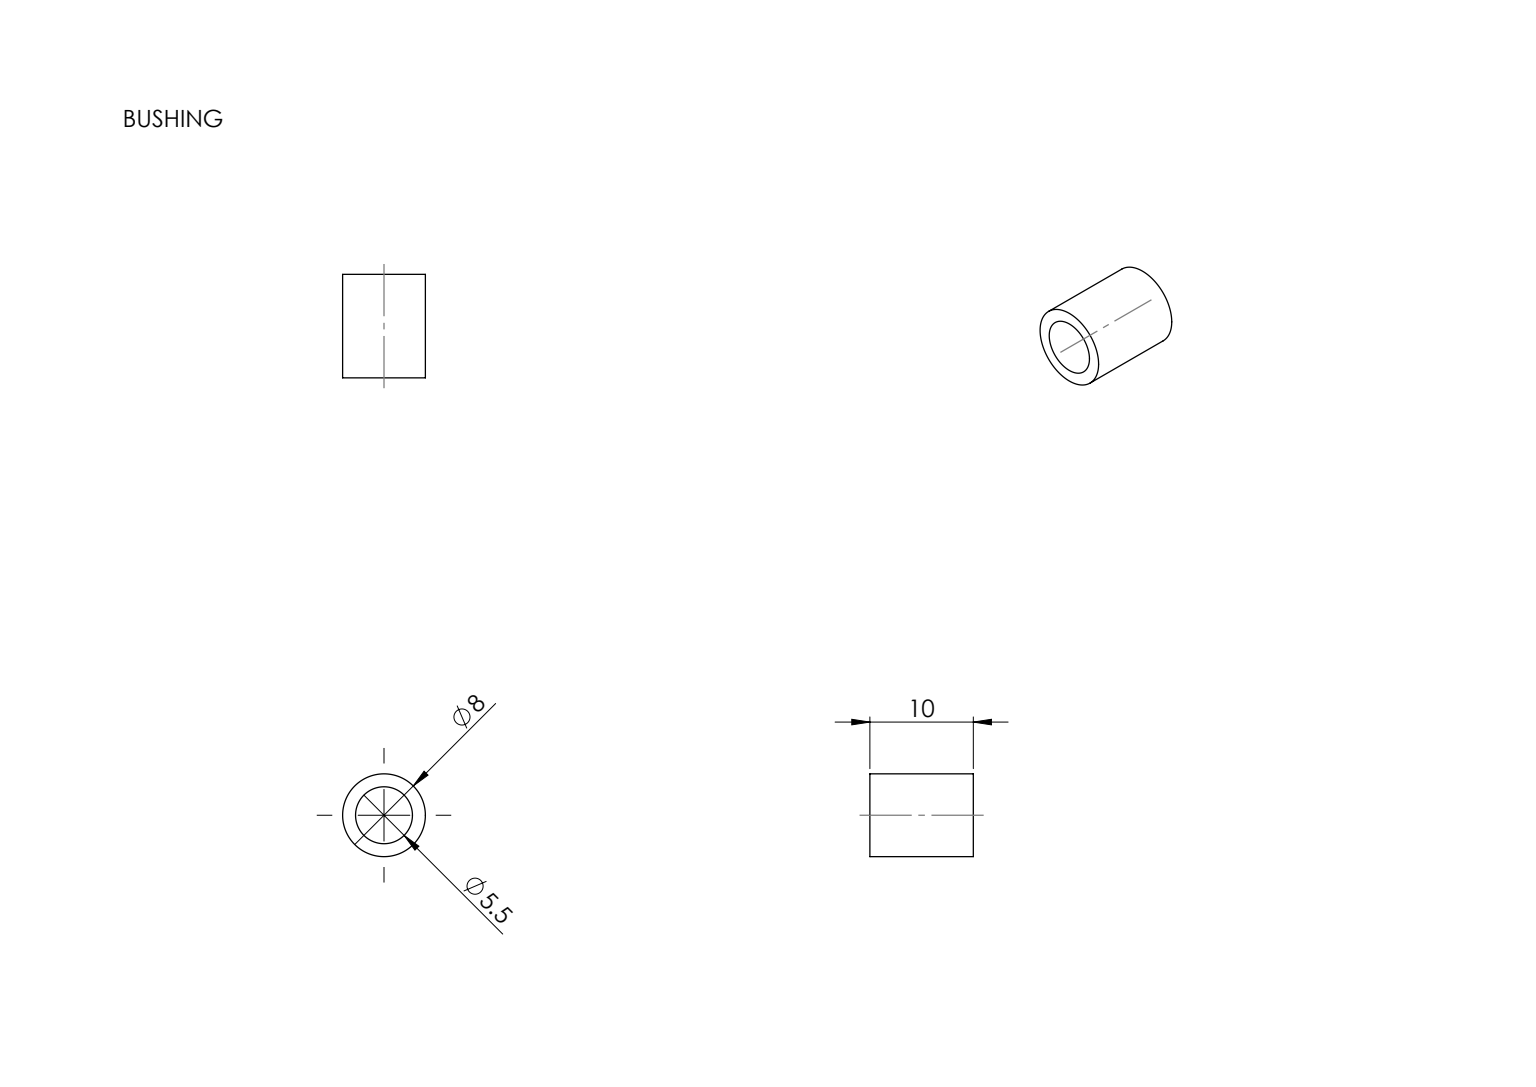
ISO-10303-21;
HEADER;
FILE_DESCRIPTION (('STEP AP214'),
    '1' );
FILE_NAME ('bushing.step',
    '2026-09-30T16:28:02',
    ( '' ),
    ( '' ),
    'SwSTEP 2.0',
    'SolidWorks 2026',
    '' );
FILE_SCHEMA (( 'AUTOMOTIVE_DESIGN' ));
ENDSEC;

DATA;
#342=ORIENTED_EDGE ( 'NONE', *, *, #14480, .T. ) ;
#400=CARTESIAN_POINT ( 'NONE',  ( -20.00000000000017053, 34.64101615137744972, 0.000000000000000000 ) ) ;
#438=VERTEX_POINT ( 'NONE', #10483 ) ;
#878=DIRECTION ( 'NONE',  ( 0.000000000000000000, 0.000000000000000000, 1.000000000000000000 ) ) ;
#913=EDGE_CURVE ( 'NONE', #9720, #12877, #3381, .T. ) ;
#981=VERTEX_POINT ( 'NONE', #7016 ) ;
#1187=EDGE_LOOP ( 'NONE', ( #17493, #27791 ) ) ;
#1368=ORIENTED_EDGE ( 'NONE', *, *, #19922, .T. ) ;
#1525=AXIS2_PLACEMENT_3D ( 'NONE', #5532, #7380, #9941 ) ;
#1531=STYLED_ITEM ( 'NONE', ( #19269 ), #18930 ) ;
#1859=DIRECTION ( 'NONE',  ( 1.000000000000000000, 0.000000000000000000, 0.000000000000000000 ) ) ;
#1982=CARTESIAN_POINT ( 'NONE',  ( -17.25000000000017053, 34.64101615137744972, 0.000000000000000000 ) ) ;
#2020=DIRECTION ( 'NONE',  ( 1.000000000000000000, 0.000000000000000000, 0.000000000000000000 ) ) ;
#2096=ORIENTED_EDGE ( 'NONE', *, *, #6742, .T. ) ;
#2144=ADVANCED_FACE ( 'NONE', ( #16550 ), #18690, .F. ) ;
#2480=ORIENTED_EDGE ( 'NONE', *, *, #3241, .T. ) ;
#2579=CARTESIAN_POINT ( 'NONE',  ( -20.00000000000017053, 34.64101615137744972, -10.00000000000000000 ) ) ;
#2867=ORIENTED_EDGE ( 'NONE', *, *, #3241, .F. ) ;
#2977=FILL_AREA_STYLE ('',( #14981 ) ) ;
#3005=EDGE_CURVE ( 'NONE', #981, #10296, #20850, .T. ) ;
#3096=SURFACE_STYLE_FILL_AREA ( #12821 ) ;
#3241=EDGE_CURVE ( 'NONE', #18375, #23025, #19355, .T. ) ;
#3259=LINE ( 'NONE', #16820, #11693 ) ;
#3381=CIRCLE ( 'NONE', #20420, 2.749999999999999112 ) ;
#3528=FILL_AREA_STYLE_COLOUR ( '', #18328 ) ;
#3562=( NAMED_UNIT ( * ) PLANE_ANGLE_UNIT ( ) SI_UNIT ( $, .RADIAN. ) );
#3641=APPLICATION_CONTEXT ( 'automotive_design' ) ;
#3688=DIRECTION ( 'NONE',  ( 0.000000000000000000, 0.000000000000000000, 1.000000000000000000 ) ) ;
#3857=EDGE_CURVE ( 'NONE', #438, #18375, #26915, .T. ) ;
#3951=EDGE_CURVE ( 'NONE', #438, #24310, #6435, .T. ) ;
#4027=CARTESIAN_POINT ( 'NONE',  ( -20.00000000000017053, 34.64101615137744972, 0.000000000000000000 ) ) ;
#4120=DIRECTION ( 'NONE',  ( 0.000000000000000000, 0.000000000000000000, 1.000000000000000000 ) ) ;
#4525=ORIENTED_EDGE ( 'NONE', *, *, #913, .T. ) ;
#5101=CARTESIAN_POINT ( 'NONE',  ( -20.00000000000017053, 34.64101615137744972, -10.00000000000000000 ) ) ;
#5174=STYLED_ITEM ( 'NONE', ( #10528 ), #21737 ) ;
#5411=VECTOR ( 'NONE', #8491, 1000.000000000000000 ) ;
#5435=CARTESIAN_POINT ( 'NONE',  ( 0.000000000000000000, 0.000000000000000000, 0.000000000000000000 ) ) ;
#5532=CARTESIAN_POINT ( 'NONE',  ( -20.00000000000017053, 34.64101615137744972, -10.00000000000000000 ) ) ;
#5843=ORIENTED_EDGE ( 'NONE', *, *, #6742, .F. ) ;
#6089=ADVANCED_FACE ( 'NONE', ( #9798 ), #14669, .T. ) ;
#6153=PRODUCT_DEFINITION ( 'UNKNOWN', '', #13639, #14055 ) ;
#6280=CARTESIAN_POINT ( 'NONE',  ( -24.00000000000017053, 34.64101615137744972, -10.00000000000000000 ) ) ;
#6306=CARTESIAN_POINT ( 'NONE',  ( -20.00000000000017053, 34.64101615137744972, -10.00000000000000000 ) ) ;
#6435=LINE ( 'NONE', #6280, #19995 ) ;
#6574=CARTESIAN_POINT ( 'NONE',  ( -20.00000000000017053, 34.64101615137744972, 0.000000000000000000 ) ) ;
#6742=EDGE_CURVE ( 'NONE', #9720, #981, #20386, .T. ) ;
#6759=APPLICATION_CONTEXT ( 'automotive_design' ) ;
#6882=( GEOMETRIC_REPRESENTATION_CONTEXT ( 3 ) GLOBAL_UNCERTAINTY_ASSIGNED_CONTEXT ( ( #16508 ) ) GLOBAL_UNIT_ASSIGNED_CONTEXT ( ( #14232, #3562, #21571 ) ) REPRESENTATION_CONTEXT ( 'NONE', 'WORKASPACE' ) );
#7016=CARTESIAN_POINT ( 'NONE',  ( -22.75000000000017053, 34.64101615137744972, 0.000000000000000000 ) ) ;
#7136=MECHANICAL_DESIGN_GEOMETRIC_PRESENTATION_REPRESENTATION('',(#5174),#20264);
#7284=DIRECTION ( 'NONE',  ( 1.000000000000000000, 0.000000000000000000, -0.000000000000000000 ) ) ;
#7380=DIRECTION ( 'NONE',  ( 0.000000000000000000, 0.000000000000000000, 1.000000000000000000 ) ) ;
#7562=DIRECTION ( 'NONE',  ( 1.000000000000000000, 0.000000000000000000, 0.000000000000000000 ) ) ;
#7796=SHAPE_DEFINITION_REPRESENTATION ( #24716, #18708 ) ;
#7820=ORIENTED_EDGE ( 'NONE', *, *, #3951, .F. ) ;
#7822=ORIENTED_EDGE ( 'NONE', *, *, #29687, .F. ) ;
#7937=PRODUCT_CONTEXT ( 'NONE', #3641, 'mechanical' ) ;
#7944=( NAMED_UNIT ( * ) SI_UNIT ( $, .STERADIAN. ) SOLID_ANGLE_UNIT ( ) );
#8137=CARTESIAN_POINT ( 'NONE',  ( -20.00000000000017053, 34.64101615137744972, -10.00000000000000000 ) ) ;
#8330=DIRECTION ( 'NONE',  ( 0.000000000000000000, 0.000000000000000000, 1.000000000000000000 ) ) ;
#8491=DIRECTION ( 'NONE',  ( 0.000000000000000000, 0.000000000000000000, 1.000000000000000000 ) ) ;
#8497=EDGE_CURVE ( 'NONE', #12877, #9720, #19608, .T. ) ;
#8541=ORIENTED_EDGE ( 'NONE', *, *, #29687, .T. ) ;
#8596=ORIENTED_EDGE ( 'NONE', *, *, #8497, .T. ) ;
#9132=CARTESIAN_POINT ( 'NONE',  ( -16.00000000000017053, 34.64101615137744972, -10.00000000000000000 ) ) ;
#9507=ADVANCED_FACE ( 'NONE', ( #25912, #18874 ), #28232, .T. ) ;
#9709=FACE_OUTER_BOUND ( 'NONE', #16105, .T. ) ;
#9720=VERTEX_POINT ( 'NONE', #10160 ) ;
#9798=FACE_OUTER_BOUND ( 'NONE', #13152, .T. ) ;
#9920=ORIENTED_EDGE ( 'NONE', *, *, #8497, .F. ) ;
#9941=DIRECTION ( 'NONE',  ( 1.000000000000000000, 0.000000000000000000, 0.000000000000000000 ) ) ;
#10160=CARTESIAN_POINT ( 'NONE',  ( -22.75000000000017053, 34.64101615137744972, -10.00000000000000000 ) ) ;
#10296=VERTEX_POINT ( 'NONE', #1982 ) ;
#10445=ADVANCED_FACE ( 'NONE', ( #9709 ), #14735, .F. ) ;
#10446=DIRECTION ( 'NONE',  ( 1.000000000000000000, 0.000000000000000000, 0.000000000000000000 ) ) ;
#10483=CARTESIAN_POINT ( 'NONE',  ( -24.00000000000017053, 34.64101615137744972, -10.00000000000000000 ) ) ;
#10528=PRESENTATION_STYLE_ASSIGNMENT (( #22133 ) ) ;
#10573=DIRECTION ( 'NONE',  ( 0.000000000000000000, 0.000000000000000000, 1.000000000000000000 ) ) ;
#10667=VECTOR ( 'NONE', #8330, 1000.000000000000000 ) ;
#10824=CYLINDRICAL_SURFACE ( 'NONE', #17451, 4.000000000000000000 ) ;
#11373=EDGE_LOOP ( 'NONE', ( #25982, #342 ) ) ;
#11394=AXIS2_PLACEMENT_3D ( 'NONE', #16463, #28112, #14009 ) ;
#11419=CARTESIAN_POINT ( 'NONE',  ( -20.00000000000017053, 34.64101615137744972, -10.00000000000000000 ) ) ;
#11693=VECTOR ( 'NONE', #28776, 1000.000000000000000 ) ;
#12254=SURFACE_STYLE_FILL_AREA ( #2977 ) ;
#12542=ORIENTED_EDGE ( 'NONE', *, *, #22205, .T. ) ;
#12765=CARTESIAN_POINT ( 'NONE',  ( -16.00000000000017053, 34.64101615137744972, 0.000000000000000000 ) ) ;
#12821=FILL_AREA_STYLE ('',( #3528 ) ) ;
#12877=VERTEX_POINT ( 'NONE', #22678 ) ;
#12989=DIRECTION ( 'NONE',  ( 0.000000000000000000, 0.000000000000000000, 1.000000000000000000 ) ) ;
#13152=EDGE_LOOP ( 'NONE', ( #1368, #17944, #29477, #2867 ) ) ;
#13190=AXIS2_PLACEMENT_3D ( 'NONE', #5435, #19606, #10446 ) ;
#13279=DIRECTION ( 'NONE',  ( 0.000000000000000000, 0.000000000000000000, 1.000000000000000000 ) ) ;
#13322=DIRECTION ( 'NONE',  ( 0.000000000000000000, 0.000000000000000000, 1.000000000000000000 ) ) ;
#13639=PRODUCT_DEFINITION_FORMATION_WITH_SPECIFIED_SOURCE ( 'ANY', '', #29395, .NOT_KNOWN. ) ;
#14009=DIRECTION ( 'NONE',  ( 1.000000000000000000, 0.000000000000000000, -0.000000000000000000 ) ) ;
#14055=PRODUCT_DEFINITION_CONTEXT ( 'detailed design', #6759, 'design' ) ;
#14232=( LENGTH_UNIT ( ) NAMED_UNIT ( * ) SI_UNIT ( .MILLI., .METRE. ) );
#14480=EDGE_CURVE ( 'NONE', #24310, #23025, #22223, .T. ) ;
#14644=EDGE_LOOP ( 'NONE', ( #23013, #19826 ) ) ;
#14669=CYLINDRICAL_SURFACE ( 'NONE', #1525, 4.000000000000000000 ) ;
#14735=CYLINDRICAL_SURFACE ( 'NONE', #29560, 2.749999999999999112 ) ;
#14980=DIRECTION ( 'NONE',  ( 0.000000000000000000, 0.000000000000000000, 1.000000000000000000 ) ) ;
#14981=FILL_AREA_STYLE_COLOUR ( '', #28864 ) ;
#15411=EDGE_CURVE ( 'NONE', #23025, #24310, #28154, .T. ) ;
#16105=EDGE_LOOP ( 'NONE', ( #24147, #2096, #22338, #7822 ) ) ;
#16164=DIRECTION ( 'NONE',  ( 1.000000000000000000, 0.000000000000000000, 0.000000000000000000 ) ) ;
#16463=CARTESIAN_POINT ( 'NONE',  ( -20.00000000000017053, 34.64101615137744972, -10.00000000000000000 ) ) ;
#16508=UNCERTAINTY_MEASURE_WITH_UNIT (LENGTH_MEASURE( 1.000000000000000082E-05 ), #14232, 'distance_accuracy_value', 'NONE');
#16550=FACE_OUTER_BOUND ( 'NONE', #26306, .T. ) ;
#16722=DIRECTION ( 'NONE',  ( 0.000000000000000000, 0.000000000000000000, 1.000000000000000000 ) ) ;
#16820=CARTESIAN_POINT ( 'NONE',  ( -17.25000000000017053, 34.64101615137744972, -10.00000000000000000 ) ) ;
#17289=CIRCLE ( 'NONE', #20206, 4.000000000000000000 ) ;
#17451=AXIS2_PLACEMENT_3D ( 'NONE', #11419, #4120, #20725 ) ;
#17493=ORIENTED_EDGE ( 'NONE', *, *, #22205, .F. ) ;
#17581=SHAPE_REPRESENTATION_RELATIONSHIP ( 'NONE' , 'NONE' ,  #18708, #18930 ) ;
#17944=ORIENTED_EDGE ( 'NONE', *, *, #3951, .T. ) ;
#17977=ORIENTED_EDGE ( 'NONE', *, *, #14480, .F. ) ;
#18081=( GEOMETRIC_REPRESENTATION_CONTEXT ( 3 ) GLOBAL_UNCERTAINTY_ASSIGNED_CONTEXT ( ( #22336 ) ) GLOBAL_UNIT_ASSIGNED_CONTEXT ( ( #24465, #22167, #26469 ) ) REPRESENTATION_CONTEXT ( 'NONE', 'WORKASPACE' ) );
#18250=CARTESIAN_POINT ( 'NONE',  ( -22.75000000000017053, 34.64101615137744972, -10.00000000000000000 ) ) ;
#18328=COLOUR_RGB ( '', 0.31764706, 0.68627451, 0.89019608) ;
#18375=VERTEX_POINT ( 'NONE', #9132 ) ;
#18378=ADVANCED_FACE ( 'NONE', ( #21349, #19059 ), #26096, .F. ) ;
#18456=CARTESIAN_POINT ( 'NONE',  ( -20.00000000000017053, 34.64101615137744972, -10.00000000000000000 ) ) ;
#18570=MECHANICAL_DESIGN_GEOMETRIC_PRESENTATION_REPRESENTATION('',(#1531),#18081);
#18614=DIRECTION ( 'NONE',  ( 1.000000000000000000, 0.000000000000000000, 0.000000000000000000 ) ) ;
#18690=CYLINDRICAL_SURFACE ( 'NONE', #24669, 2.749999999999999112 ) ;
#18708=SHAPE_REPRESENTATION ( 'bushing', ( #13190 ), #6882 ) ;
#18874=FACE_OUTER_BOUND ( 'NONE', #11373, .T. ) ;
#18930=ADVANCED_BREP_SHAPE_REPRESENTATION ( '', ( #21737, #13190 ), #6882 ) ;
#19059=FACE_OUTER_BOUND ( 'NONE', #14644, .T. ) ;
#19205=CARTESIAN_POINT ( 'NONE',  ( -16.00000000000017053, 34.64101615137744972, -10.00000000000000000 ) ) ;
#19239=( LENGTH_UNIT ( ) NAMED_UNIT ( * ) SI_UNIT ( .MILLI., .METRE. ) );
#19269=PRESENTATION_STYLE_ASSIGNMENT (( #24317 ) ) ;
#19355=LINE ( 'NONE', #19205, #10667 ) ;
#19606=DIRECTION ( 'NONE',  ( 0.000000000000000000, 0.000000000000000000, 1.000000000000000000 ) ) ;
#19608=CIRCLE ( 'NONE', #20112, 2.749999999999999112 ) ;
#19716=SURFACE_SIDE_STYLE ('',( #12254 ) ) ;
#19826=ORIENTED_EDGE ( 'NONE', *, *, #3857, .F. ) ;
#19870=DIRECTION ( 'NONE',  ( 1.000000000000000000, 0.000000000000000000, 0.000000000000000000 ) ) ;
#19922=EDGE_CURVE ( 'NONE', #18375, #438, #17289, .T. ) ;
#19995=VECTOR ( 'NONE', #3688, 1000.000000000000000 ) ;
#20112=AXIS2_PLACEMENT_3D ( 'NONE', #18456, #13279, #1859 ) ;
#20171=CARTESIAN_POINT ( 'NONE',  ( -20.00000000000017053, 34.64101615137744972, 0.000000000000000000 ) ) ;
#20206=AXIS2_PLACEMENT_3D ( 'NONE', #8137, #22335, #24939 ) ;
#20264=( GEOMETRIC_REPRESENTATION_CONTEXT ( 3 ) GLOBAL_UNCERTAINTY_ASSIGNED_CONTEXT ( ( #28160 ) ) GLOBAL_UNIT_ASSIGNED_CONTEXT ( ( #19239, #21836, #7944 ) ) REPRESENTATION_CONTEXT ( 'NONE', 'WORKASPACE' ) );
#20386=LINE ( 'NONE', #18250, #5411 ) ;
#20420=AXIS2_PLACEMENT_3D ( 'NONE', #6306, #10573, #16164 ) ;
#20725=DIRECTION ( 'NONE',  ( 1.000000000000000000, 0.000000000000000000, 0.000000000000000000 ) ) ;
#20850=CIRCLE ( 'NONE', #25749, 2.749999999999999112 ) ;
#20933=EDGE_LOOP ( 'NONE', ( #8596, #4525 ) ) ;
#20970=DIRECTION ( 'NONE',  ( 0.000000000000000000, 0.000000000000000000, 1.000000000000000000 ) ) ;
#21349=FACE_BOUND ( 'NONE', #20933, .T. ) ;
#21468=DIRECTION ( 'NONE',  ( 0.000000000000000000, 0.000000000000000000, 1.000000000000000000 ) ) ;
#21537=SURFACE_SIDE_STYLE ('',( #3096 ) ) ;
#21571=( NAMED_UNIT ( * ) SI_UNIT ( $, .STERADIAN. ) SOLID_ANGLE_UNIT ( ) );
#21737=MANIFOLD_SOLID_BREP ( 'Extrude-Thin1', #28269 ) ;
#21809=ORIENTED_EDGE ( 'NONE', *, *, #3857, .T. ) ;
#21836=( NAMED_UNIT ( * ) PLANE_ANGLE_UNIT ( ) SI_UNIT ( $, .RADIAN. ) );
#22013=CARTESIAN_POINT ( 'NONE',  ( -24.00000000000017053, 34.64101615137744972, 0.000000000000000000 ) ) ;
#22133=SURFACE_STYLE_USAGE ( .BOTH. , #21537 ) ;
#22160=EDGE_LOOP ( 'NONE', ( #7820, #21809, #2480, #17977 ) ) ;
#22167=( NAMED_UNIT ( * ) PLANE_ANGLE_UNIT ( ) SI_UNIT ( $, .RADIAN. ) );
#22205=EDGE_CURVE ( 'NONE', #10296, #981, #29126, .T. ) ;
#22223=CIRCLE ( 'NONE', #23205, 4.000000000000000000 ) ;
#22335=DIRECTION ( 'NONE',  ( 0.000000000000000000, 0.000000000000000000, 1.000000000000000000 ) ) ;
#22336=UNCERTAINTY_MEASURE_WITH_UNIT (LENGTH_MEASURE( 1.000000000000000082E-05 ), #24465, 'distance_accuracy_value', 'NONE');
#22338=ORIENTED_EDGE ( 'NONE', *, *, #3005, .T. ) ;
#22502=DIRECTION ( 'NONE',  ( 1.000000000000000000, 0.000000000000000000, 0.000000000000000000 ) ) ;
#22589=FACE_OUTER_BOUND ( 'NONE', #22160, .T. ) ;
#22610=CARTESIAN_POINT ( 'NONE',  ( -20.00000000000017053, 34.64101615137744972, -10.00000000000000000 ) ) ;
#22678=CARTESIAN_POINT ( 'NONE',  ( -17.25000000000017053, 34.64101615137744972, -10.00000000000000000 ) ) ;
#23013=ORIENTED_EDGE ( 'NONE', *, *, #19922, .F. ) ;
#23025=VERTEX_POINT ( 'NONE', #12765 ) ;
#23205=AXIS2_PLACEMENT_3D ( 'NONE', #400, #16722, #7562 ) ;
#24147=ORIENTED_EDGE ( 'NONE', *, *, #913, .F. ) ;
#24310=VERTEX_POINT ( 'NONE', #22013 ) ;
#24317=SURFACE_STYLE_USAGE ( .BOTH. , #19716 ) ;
#24386=AXIS2_PLACEMENT_3D ( 'NONE', #22610, #12989, #2020 ) ;
#24465=( LENGTH_UNIT ( ) NAMED_UNIT ( * ) SI_UNIT ( .MILLI., .METRE. ) );
#24669=AXIS2_PLACEMENT_3D ( 'NONE', #5101, #20970, #27891 ) ;
#24716=PRODUCT_DEFINITION_SHAPE ( 'NONE', 'NONE',  #6153 ) ;
#24939=DIRECTION ( 'NONE',  ( 1.000000000000000000, 0.000000000000000000, 0.000000000000000000 ) ) ;
#25341=DIRECTION ( 'NONE',  ( 0.000000000000000000, 0.000000000000000000, 1.000000000000000000 ) ) ;
#25676=AXIS2_PLACEMENT_3D ( 'NONE', #4027, #13322, #22502 ) ;
#25749=AXIS2_PLACEMENT_3D ( 'NONE', #6574, #25341, #18614 ) ;
#25912=FACE_BOUND ( 'NONE', #1187, .T. ) ;
#25982=ORIENTED_EDGE ( 'NONE', *, *, #15411, .T. ) ;
#26096=PLANE ( 'NONE',  #11394 ) ;
#26306=EDGE_LOOP ( 'NONE', ( #5843, #9920, #8541, #12542 ) ) ;
#26469=( NAMED_UNIT ( * ) SI_UNIT ( $, .STERADIAN. ) SOLID_ANGLE_UNIT ( ) );
#26784=ADVANCED_FACE ( 'NONE', ( #22589 ), #10824, .T. ) ;
#26915=CIRCLE ( 'NONE', #24386, 4.000000000000000000 ) ;
#27791=ORIENTED_EDGE ( 'NONE', *, *, #3005, .F. ) ;
#27891=DIRECTION ( 'NONE',  ( 1.000000000000000000, 0.000000000000000000, 0.000000000000000000 ) ) ;
#28112=DIRECTION ( 'NONE',  ( 0.000000000000000000, 0.000000000000000000, 1.000000000000000000 ) ) ;
#28154=CIRCLE ( 'NONE', #30112, 4.000000000000000000 ) ;
#28160=UNCERTAINTY_MEASURE_WITH_UNIT (LENGTH_MEASURE( 1.000000000000000082E-05 ), #19239, 'distance_accuracy_value', 'NONE');
#28232=PLANE ( 'NONE',  #29800 ) ;
#28269=CLOSED_SHELL ( 'NONE', ( #10445, #6089, #26784, #18378, #9507, #2144 ) ) ;
#28391=DIRECTION ( 'NONE',  ( 1.000000000000000000, 0.000000000000000000, 0.000000000000000000 ) ) ;
#28681=CARTESIAN_POINT ( 'NONE',  ( -20.00000000000017053, 34.64101615137744972, 0.000000000000000000 ) ) ;
#28776=DIRECTION ( 'NONE',  ( 0.000000000000000000, 0.000000000000000000, 1.000000000000000000 ) ) ;
#28864=COLOUR_RGB ( '', 0.31764706, 0.68627451, 0.89019608) ;
#29126=CIRCLE ( 'NONE', #25676, 2.749999999999999112 ) ;
#29395=PRODUCT ( 'bushing', 'bushing', '', ( #7937 ) ) ;
#29477=ORIENTED_EDGE ( 'NONE', *, *, #15411, .F. ) ;
#29560=AXIS2_PLACEMENT_3D ( 'NONE', #2579, #878, #28391 ) ;
#29687=EDGE_CURVE ( 'NONE', #12877, #10296, #3259, .T. ) ;
#29800=AXIS2_PLACEMENT_3D ( 'NONE', #28681, #21468, #7284 ) ;
#30112=AXIS2_PLACEMENT_3D ( 'NONE', #20171, #14980, #19870 ) ;
ENDSEC;
END-ISO-10303-21;
